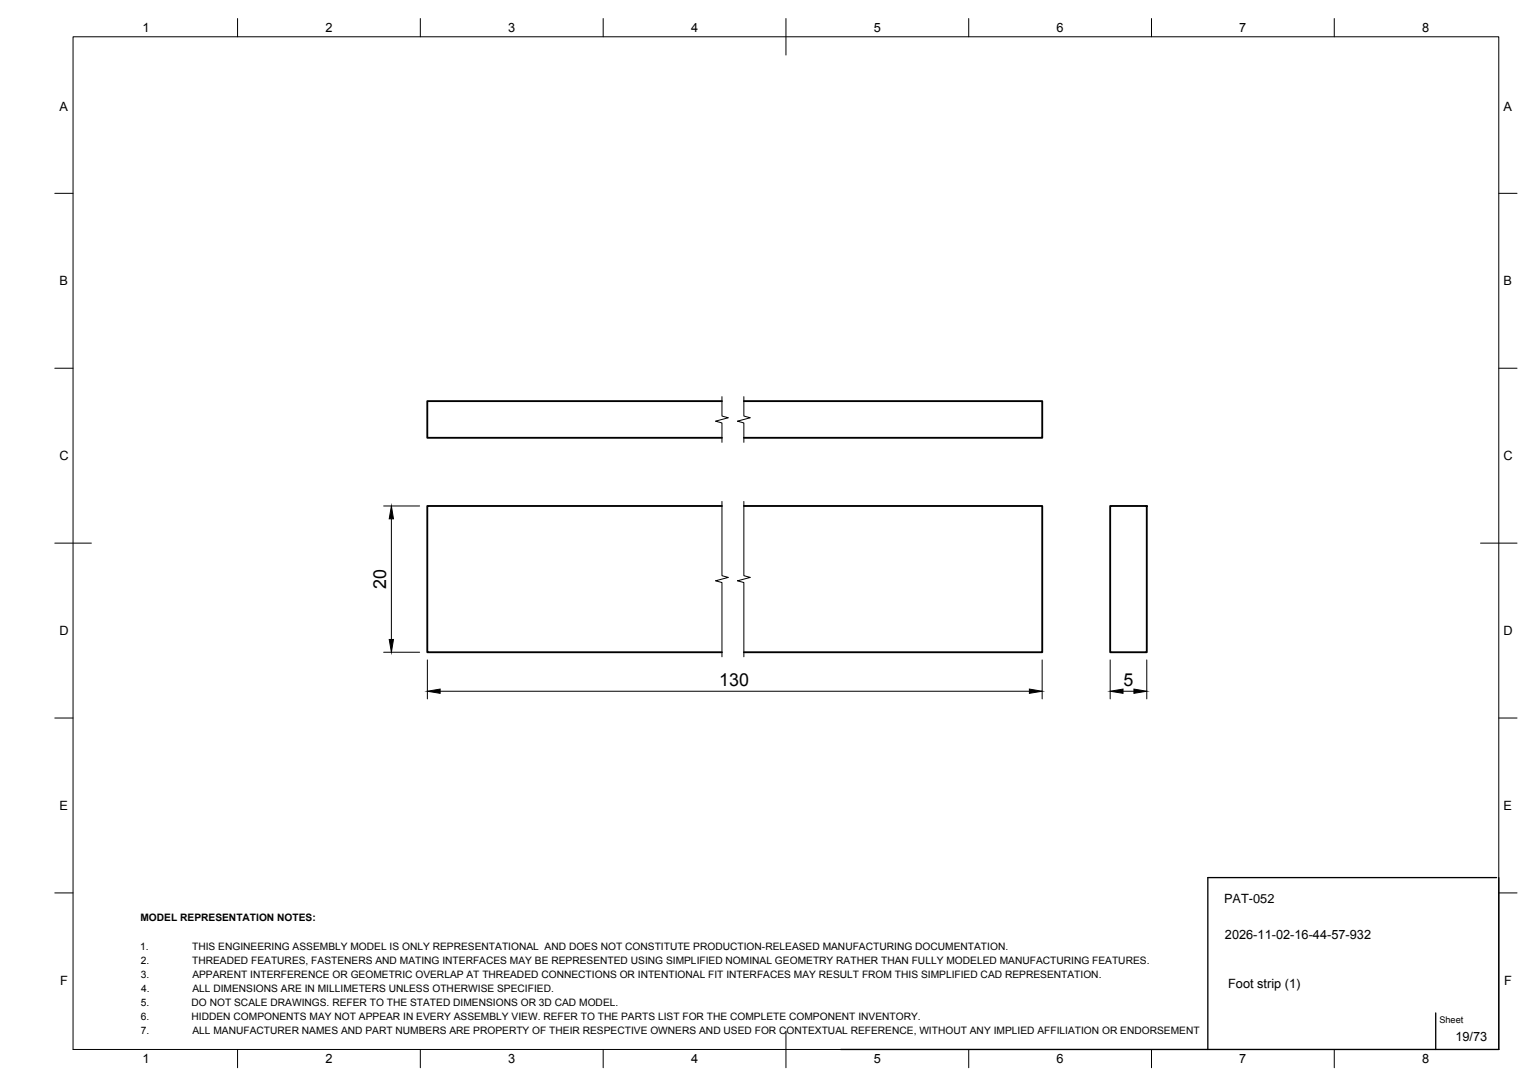
ISO-10303-21;
HEADER;
/* Generated by software containing ST-Developer
 * from STEP Tools, Inc. (www.steptools.com) 
 */

FILE_DESCRIPTION(
/* description */ ('Hand-crank gear train demonstrator'),
/* implementation_level */ '2;1');

FILE_NAME(
/* name */ 'Foot strip (1).step',
/* time_stamp */ '2026-10-28T03:22:13-07:00',
/* author */ (''),
/* organization */ (''),
/* preprocessor_version */ 'ST-DEVELOPER v20.2',
/* originating_system */ 'Autodesk Translation Framework v15.17.0.0',
/* authorisation */ '');

FILE_SCHEMA (('AUTOMOTIVE_DESIGN { 1 0 10303 214 3 1 1 }'));
ENDSEC;

DATA;
#10=MECHANICAL_DESIGN_GEOMETRIC_PRESENTATION_REPRESENTATION('',(#1230),#62758);
#1087=SHAPE_REPRESENTATION_RELATIONSHIP('SRR','None',#63061,#1151);
#1151=ADVANCED_BREP_SHAPE_REPRESENTATION('',(#1307),#62715);
#1230=STYLED_ITEM('',(#63448),#1307);
#1307=MANIFOLD_SOLID_BREP('Body1',#16412);
#1865=PLANE('',#17938);
#1866=PLANE('',#17939);
#1867=PLANE('',#17940);
#1868=PLANE('',#17941);
#1869=PLANE('',#17942);
#1870=PLANE('',#17943);
#2523=FACE_OUTER_BOUND('',#3657,.T.);
#2524=FACE_OUTER_BOUND('',#3658,.T.);
#2525=FACE_OUTER_BOUND('',#3659,.T.);
#2526=FACE_OUTER_BOUND('',#3660,.T.);
#2527=FACE_OUTER_BOUND('',#3661,.T.);
#2528=FACE_OUTER_BOUND('',#3662,.T.);
#3657=EDGE_LOOP('',(#12619,#12620,#12621,#12622));
#3658=EDGE_LOOP('',(#12623,#12624,#12625,#12626));
#3659=EDGE_LOOP('',(#12627,#12628,#12629,#12630));
#3660=EDGE_LOOP('',(#12631,#12632,#12633,#12634));
#3661=EDGE_LOOP('',(#12635,#12636,#12637,#12638));
#3662=EDGE_LOOP('',(#12639,#12640,#12641,#12642));
#4807=LINE('',#25887,#5939);
#4808=LINE('',#25889,#5940);
#4809=LINE('',#25891,#5941);
#4810=LINE('',#25892,#5942);
#4811=LINE('',#25895,#5943);
#4812=LINE('',#25897,#5944);
#4813=LINE('',#25898,#5945);
#4814=LINE('',#25901,#5946);
#4815=LINE('',#25903,#5947);
#4816=LINE('',#25904,#5948);
#4817=LINE('',#25906,#5949);
#4818=LINE('',#25907,#5950);
#5939=VECTOR('',#20914,1.);
#5940=VECTOR('',#20915,1.);
#5941=VECTOR('',#20916,1.);
#5942=VECTOR('',#20917,1.);
#5943=VECTOR('',#20920,1.);
#5944=VECTOR('',#20921,1.);
#5945=VECTOR('',#20922,1.);
#5946=VECTOR('',#20925,1.);
#5947=VECTOR('',#20926,1.);
#5948=VECTOR('',#20927,1.);
#5949=VECTOR('',#20930,1.);
#5950=VECTOR('',#20931,1.);
#7822=VERTEX_POINT('',#25885);
#7823=VERTEX_POINT('',#25886);
#7824=VERTEX_POINT('',#25888);
#7825=VERTEX_POINT('',#25890);
#7826=VERTEX_POINT('',#25894);
#7827=VERTEX_POINT('',#25896);
#7828=VERTEX_POINT('',#25900);
#7829=VERTEX_POINT('',#25902);
#9561=EDGE_CURVE('',#7822,#7823,#4807,.T.);
#9562=EDGE_CURVE('',#7823,#7824,#4808,.T.);
#9563=EDGE_CURVE('',#7825,#7824,#4809,.T.);
#9564=EDGE_CURVE('',#7822,#7825,#4810,.T.);
#9565=EDGE_CURVE('',#7826,#7822,#4811,.T.);
#9566=EDGE_CURVE('',#7827,#7825,#4812,.T.);
#9567=EDGE_CURVE('',#7826,#7827,#4813,.T.);
#9568=EDGE_CURVE('',#7828,#7826,#4814,.T.);
#9569=EDGE_CURVE('',#7829,#7827,#4815,.T.);
#9570=EDGE_CURVE('',#7828,#7829,#4816,.T.);
#9571=EDGE_CURVE('',#7823,#7828,#4817,.T.);
#9572=EDGE_CURVE('',#7824,#7829,#4818,.T.);
#12619=ORIENTED_EDGE('',*,*,#9561,.T.);
#12620=ORIENTED_EDGE('',*,*,#9562,.T.);
#12621=ORIENTED_EDGE('',*,*,#9563,.F.);
#12622=ORIENTED_EDGE('',*,*,#9564,.F.);
#12623=ORIENTED_EDGE('',*,*,#9565,.T.);
#12624=ORIENTED_EDGE('',*,*,#9564,.T.);
#12625=ORIENTED_EDGE('',*,*,#9566,.F.);
#12626=ORIENTED_EDGE('',*,*,#9567,.F.);
#12627=ORIENTED_EDGE('',*,*,#9568,.T.);
#12628=ORIENTED_EDGE('',*,*,#9567,.T.);
#12629=ORIENTED_EDGE('',*,*,#9569,.F.);
#12630=ORIENTED_EDGE('',*,*,#9570,.F.);
#12631=ORIENTED_EDGE('',*,*,#9571,.T.);
#12632=ORIENTED_EDGE('',*,*,#9570,.T.);
#12633=ORIENTED_EDGE('',*,*,#9572,.F.);
#12634=ORIENTED_EDGE('',*,*,#9562,.F.);
#12635=ORIENTED_EDGE('',*,*,#9572,.T.);
#12636=ORIENTED_EDGE('',*,*,#9569,.T.);
#12637=ORIENTED_EDGE('',*,*,#9566,.T.);
#12638=ORIENTED_EDGE('',*,*,#9563,.T.);
#12639=ORIENTED_EDGE('',*,*,#9571,.F.);
#12640=ORIENTED_EDGE('',*,*,#9561,.F.);
#12641=ORIENTED_EDGE('',*,*,#9565,.F.);
#12642=ORIENTED_EDGE('',*,*,#9568,.F.);
#15833=ADVANCED_FACE('',(#2523),#1865,.T.);
#15834=ADVANCED_FACE('',(#2524),#1866,.T.);
#15835=ADVANCED_FACE('',(#2525),#1867,.T.);
#15836=ADVANCED_FACE('',(#2526),#1868,.T.);
#15837=ADVANCED_FACE('',(#2527),#1869,.T.);
#15838=ADVANCED_FACE('',(#2528),#1870,.F.);
#16412=CLOSED_SHELL('',(#15833,#15834,#15835,#15836,#15837,#15838));
#17937=AXIS2_PLACEMENT_3D('',#25883,#20910,#20911);
#17938=AXIS2_PLACEMENT_3D('',#25884,#20912,#20913);
#17939=AXIS2_PLACEMENT_3D('',#25893,#20918,#20919);
#17940=AXIS2_PLACEMENT_3D('',#25899,#20923,#20924);
#17941=AXIS2_PLACEMENT_3D('',#25905,#20928,#20929);
#17942=AXIS2_PLACEMENT_3D('',#25908,#20932,#20933);
#17943=AXIS2_PLACEMENT_3D('',#25909,#20934,#20935);
#20910=DIRECTION('axis',(0.,0.,1.));
#20911=DIRECTION('refdir',(1.,0.,0.));
#20912=DIRECTION('center_axis',(0.,1.,0.));
#20913=DIRECTION('ref_axis',(-1.,0.,0.));
#20914=DIRECTION('',(-1.,0.,0.));
#20915=DIRECTION('',(0.,0.,1.));
#20916=DIRECTION('',(-1.,0.,0.));
#20917=DIRECTION('',(0.,0.,1.));
#20918=DIRECTION('center_axis',(1.,0.,0.));
#20919=DIRECTION('ref_axis',(0.,1.,0.));
#20920=DIRECTION('',(0.,1.,0.));
#20921=DIRECTION('',(0.,1.,0.));
#20922=DIRECTION('',(0.,0.,1.));
#20923=DIRECTION('center_axis',(0.,-1.,0.));
#20924=DIRECTION('ref_axis',(1.,0.,0.));
#20925=DIRECTION('',(1.,0.,0.));
#20926=DIRECTION('',(1.,0.,0.));
#20927=DIRECTION('',(0.,0.,1.));
#20928=DIRECTION('center_axis',(-1.,0.,0.));
#20929=DIRECTION('ref_axis',(0.,-1.,0.));
#20930=DIRECTION('',(0.,-1.,0.));
#20931=DIRECTION('',(0.,-1.,0.));
#20932=DIRECTION('center_axis',(0.,0.,1.));
#20933=DIRECTION('ref_axis',(1.,0.,0.));
#20934=DIRECTION('center_axis',(0.,0.,1.));
#20935=DIRECTION('ref_axis',(1.,0.,0.));
#25883=CARTESIAN_POINT('',(0.,0.,0.));
#25884=CARTESIAN_POINT('Origin',(24.,6.5,-0.5));
#25885=CARTESIAN_POINT('',(24.,6.5,-0.5));
#25886=CARTESIAN_POINT('',(22.,6.5,-0.5));
#25887=CARTESIAN_POINT('',(24.,6.5,-0.5));
#25888=CARTESIAN_POINT('',(22.,6.5,0.));
#25889=CARTESIAN_POINT('',(22.,6.5,-0.5));
#25890=CARTESIAN_POINT('',(24.,6.5,0.));
#25891=CARTESIAN_POINT('',(24.,6.5,0.));
#25892=CARTESIAN_POINT('',(24.,6.5,-0.5));
#25893=CARTESIAN_POINT('Origin',(24.,-6.5,-0.5));
#25894=CARTESIAN_POINT('',(24.,-6.5,-0.5));
#25895=CARTESIAN_POINT('',(24.,-6.5,-0.5));
#25896=CARTESIAN_POINT('',(24.,-6.5,0.));
#25897=CARTESIAN_POINT('',(24.,-6.5,0.));
#25898=CARTESIAN_POINT('',(24.,-6.5,-0.5));
#25899=CARTESIAN_POINT('Origin',(22.,-6.5,-0.5));
#25900=CARTESIAN_POINT('',(22.,-6.5,-0.5));
#25901=CARTESIAN_POINT('',(22.,-6.5,-0.5));
#25902=CARTESIAN_POINT('',(22.,-6.5,0.));
#25903=CARTESIAN_POINT('',(22.,-6.5,0.));
#25904=CARTESIAN_POINT('',(22.,-6.5,-0.5));
#25905=CARTESIAN_POINT('Origin',(22.,6.5,-0.5));
#25906=CARTESIAN_POINT('',(22.,6.5,-0.5));
#25907=CARTESIAN_POINT('',(22.,6.5,0.));
#25908=CARTESIAN_POINT('Origin',(23.,0.,0.));
#25909=CARTESIAN_POINT('Origin',(23.,0.,-0.5));
#62641=UNCERTAINTY_MEASURE_WITH_UNIT(LENGTH_MEASURE(0.001),#62759,
'DISTANCE_ACCURACY_VALUE',
'Maximum model space distance between geometric entities at asserted c
onnectivities');
#62684=UNCERTAINTY_MEASURE_WITH_UNIT(LENGTH_MEASURE(0.001),#62759,
'DISTANCE_ACCURACY_VALUE',
'Maximum model space distance between geometric entities at asserted c
onnectivities');
#62715=(
GEOMETRIC_REPRESENTATION_CONTEXT(3)
GLOBAL_UNCERTAINTY_ASSIGNED_CONTEXT((#62641))
GLOBAL_UNIT_ASSIGNED_CONTEXT((#62759,#62761,#62762))
REPRESENTATION_CONTEXT('','3D')
);
#62758=(
GEOMETRIC_REPRESENTATION_CONTEXT(3)
GLOBAL_UNCERTAINTY_ASSIGNED_CONTEXT((#62684))
GLOBAL_UNIT_ASSIGNED_CONTEXT((#62759,#62761,#62762))
REPRESENTATION_CONTEXT('','3D')
);
#62759=(
LENGTH_UNIT()
NAMED_UNIT(*)
SI_UNIT(.CENTI.,.METRE.)
);
#62761=(
NAMED_UNIT(*)
PLANE_ANGLE_UNIT()
SI_UNIT($,.RADIAN.)
);
#62762=(
NAMED_UNIT(*)
SI_UNIT($,.STERADIAN.)
SOLID_ANGLE_UNIT()
);
#62793=SHAPE_DEFINITION_REPRESENTATION(#62876,#63061);
#62876=PRODUCT_DEFINITION_SHAPE('',$,#63135);
#63061=SHAPE_REPRESENTATION('',(#17937),#62715);
#63104=PRODUCT_DEFINITION_CONTEXT('part definition',#63325,'design');
#63135=PRODUCT_DEFINITION('Foot strip (1)','Foot strip (1)',#63208,#63104);
#63208=PRODUCT_DEFINITION_FORMATION('',$,#63357);
#63325=APPLICATION_CONTEXT(
'Core Data for Automotive Mechanical Design Process');
#63326=PRODUCT_CONTEXT('part definition',#63325,'mechanical');
#63357=PRODUCT('Foot strip (1)','Foot strip (1)','Foot strip (1)',(#63326));
#63442=COLOUR_RGB('Light Blue',0.38,0.62,0.78);
#63443=FILL_AREA_STYLE_COLOUR('',#63442);
#63444=FILL_AREA_STYLE('',(#63443));
#63445=SURFACE_STYLE_FILL_AREA(#63444);
#63446=SURFACE_SIDE_STYLE('',(#63445));
#63447=SURFACE_STYLE_USAGE(.BOTH.,#63446);
#63448=PRESENTATION_STYLE_ASSIGNMENT((#63447));
ENDSEC;
END-ISO-10303-21;
